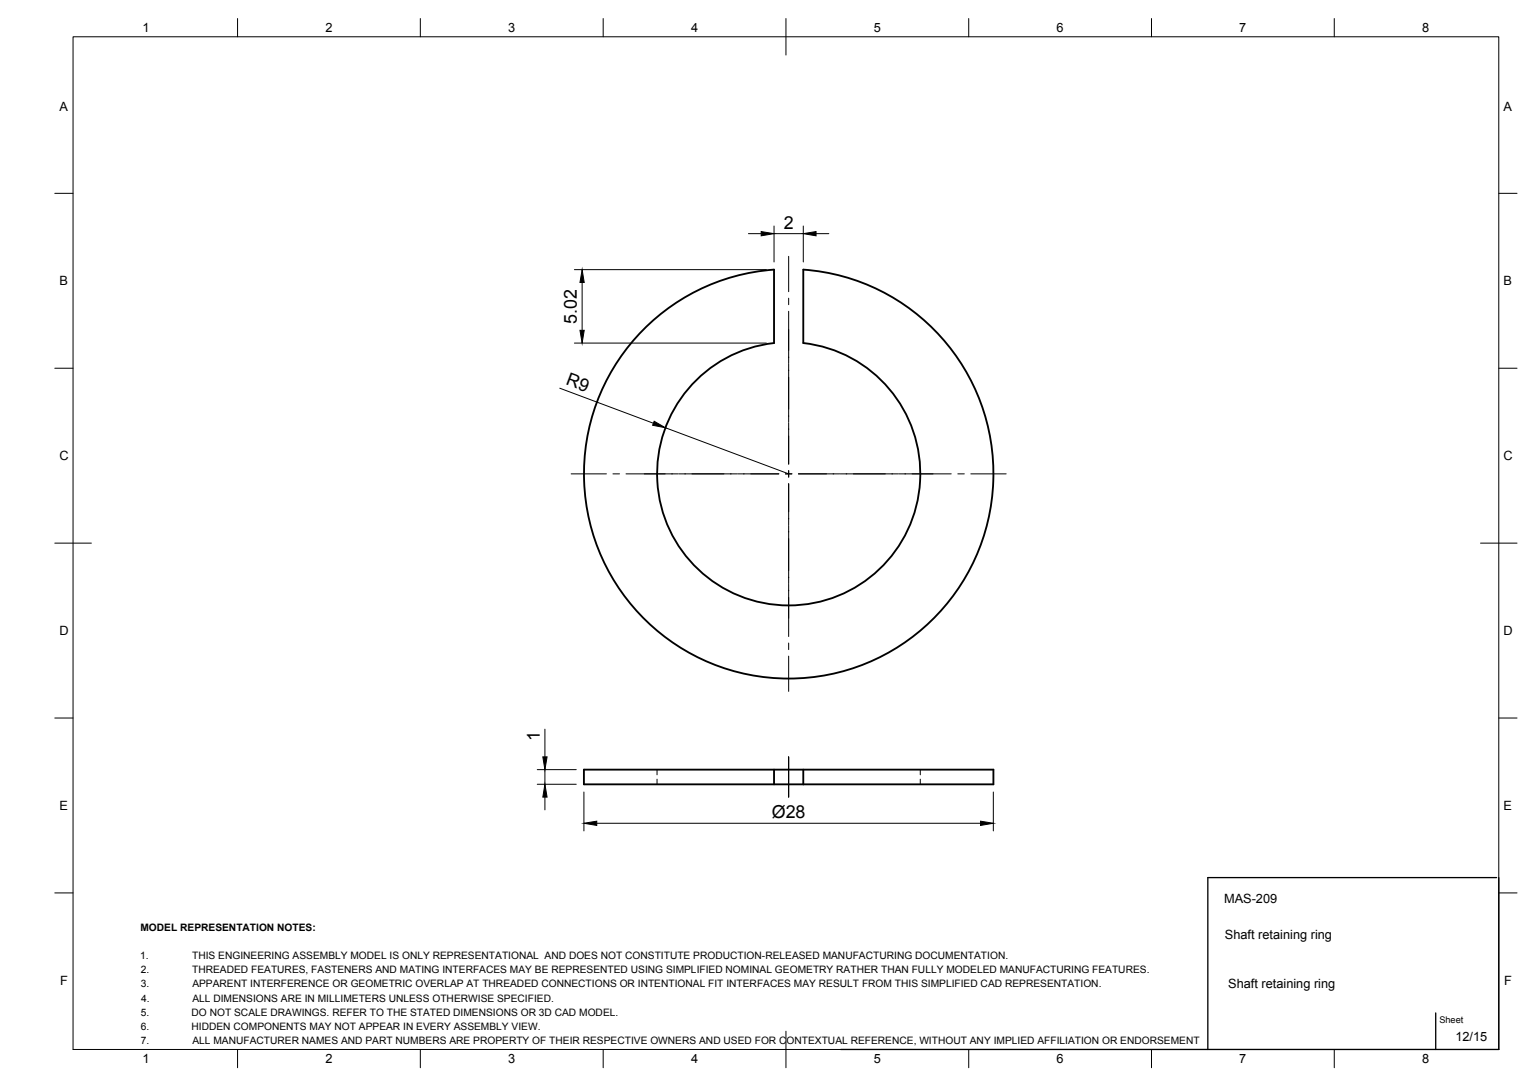
ISO-10303-21;
HEADER;
/* Generated by software containing ST-Developer
 * from STEP Tools, Inc. (www.steptools.com) 
 */

FILE_DESCRIPTION(
/* description */ ('Independent bearing-supported roller-ramp one-way clutch. Six logarit
hmic ramps with plain solid rollers, sprung guided plungers, native Co
il variants, removable shared keepers, rounded parallel key, shaft wit
h complete retaining lips, bronze journal/thrust support and bolted co
vers. Native rotor, roller planar/spin and plunger joints permit manua
l geometric engaged/released inspection. Automatic frictional torque s
witching/contact dynamics are not simulated; no capacity, hardness, fi
t, lubrication, speed, force or life rating. External input driver/cou
pling/anchors outside assembly.'),
/* implementation_level */ '2;1');

FILE_NAME(
/* name */ 'Shaft retaining ring.step',
/* time_stamp */ '2026-11-08T07:04:38-08:00',
/* author */ (''),
/* organization */ (''),
/* preprocessor_version */ 'ST-DEVELOPER v20.2',
/* originating_system */ 'Autodesk Translation Framework v15.17.0.0',
/* authorisation */ '');

FILE_SCHEMA (('AUTOMOTIVE_DESIGN { 1 0 10303 214 3 1 1 }'));
ENDSEC;

DATA;
#10=MECHANICAL_DESIGN_GEOMETRIC_PRESENTATION_REPRESENTATION('',(#311),#99526);
#279=SHAPE_REPRESENTATION_RELATIONSHIP('SRR','None',#99636,#295);
#295=ADVANCED_BREP_SHAPE_REPRESENTATION('',(#327),#99521);
#311=STYLED_ITEM('',(#99722),#327);
#327=MANIFOLD_SOLID_BREP('Body1',#18281);
#585=PLANE('',#19622);
#586=PLANE('',#19623);
#587=PLANE('',#19624);
#588=PLANE('',#19631);
#1578=FACE_OUTER_BOUND('',#2679,.T.);
#1579=FACE_OUTER_BOUND('',#2680,.T.);
#1580=FACE_OUTER_BOUND('',#2681,.T.);
#1581=FACE_OUTER_BOUND('',#2682,.T.);
#1582=FACE_OUTER_BOUND('',#2683,.T.);
#1583=FACE_OUTER_BOUND('',#2684,.T.);
#2679=EDGE_LOOP('',(#16056,#16057,#16058,#16059));
#2680=EDGE_LOOP('',(#16060,#16061,#16062,#16063));
#2681=EDGE_LOOP('',(#16064,#16065,#16066,#16067));
#2682=EDGE_LOOP('',(#16068,#16069,#16070,#16071));
#2683=EDGE_LOOP('',(#16072,#16073,#16074,#16075));
#2684=EDGE_LOOP('',(#16076,#16077,#16078,#16079));
#3088=CIRCLE('',#19625,14.);
#3089=CIRCLE('',#19626,9.);
#3090=CIRCLE('',#19628,9.);
#3091=CIRCLE('',#19630,14.);
#5436=LINE('',#94898,#6340);
#5437=LINE('',#94900,#6341);
#5438=LINE('',#94902,#6342);
#5439=LINE('',#94903,#6343);
#5440=LINE('',#94907,#6344);
#5441=LINE('',#94909,#6345);
#5442=LINE('',#94911,#6346);
#5443=LINE('',#94912,#6347);
#6340=VECTOR('',#22925,10.);
#6341=VECTOR('',#22926,10.);
#6342=VECTOR('',#22927,10.);
#6343=VECTOR('',#22928,10.);
#6344=VECTOR('',#22931,10.);
#6345=VECTOR('',#22932,10.);
#6346=VECTOR('',#22933,10.);
#6347=VECTOR('',#22934,10.);
#8103=VERTEX_POINT('',#94896);
#8104=VERTEX_POINT('',#94897);
#8105=VERTEX_POINT('',#94899);
#8106=VERTEX_POINT('',#94901);
#8107=VERTEX_POINT('',#94905);
#8108=VERTEX_POINT('',#94906);
#8109=VERTEX_POINT('',#94908);
#8110=VERTEX_POINT('',#94910);
#10780=EDGE_CURVE('',#8103,#8104,#5436,.T.);
#10781=EDGE_CURVE('',#8105,#8103,#5437,.T.);
#10782=EDGE_CURVE('',#8106,#8105,#5438,.T.);
#10783=EDGE_CURVE('',#8104,#8106,#5439,.T.);
#10784=EDGE_CURVE('',#8107,#8108,#5440,.T.);
#10785=EDGE_CURVE('',#8109,#8107,#5441,.T.);
#10786=EDGE_CURVE('',#8110,#8109,#5442,.T.);
#10787=EDGE_CURVE('',#8108,#8110,#5443,.T.);
#10788=EDGE_CURVE('',#8105,#8110,#3088,.T.);
#10789=EDGE_CURVE('',#8108,#8103,#3089,.T.);
#10790=EDGE_CURVE('',#8107,#8104,#3090,.T.);
#10791=EDGE_CURVE('',#8106,#8109,#3091,.T.);
#16056=ORIENTED_EDGE('',*,*,#10780,.F.);
#16057=ORIENTED_EDGE('',*,*,#10781,.F.);
#16058=ORIENTED_EDGE('',*,*,#10782,.F.);
#16059=ORIENTED_EDGE('',*,*,#10783,.F.);
#16060=ORIENTED_EDGE('',*,*,#10784,.F.);
#16061=ORIENTED_EDGE('',*,*,#10785,.F.);
#16062=ORIENTED_EDGE('',*,*,#10786,.F.);
#16063=ORIENTED_EDGE('',*,*,#10787,.F.);
#16064=ORIENTED_EDGE('',*,*,#10787,.T.);
#16065=ORIENTED_EDGE('',*,*,#10788,.F.);
#16066=ORIENTED_EDGE('',*,*,#10781,.T.);
#16067=ORIENTED_EDGE('',*,*,#10789,.F.);
#16068=ORIENTED_EDGE('',*,*,#10784,.T.);
#16069=ORIENTED_EDGE('',*,*,#10789,.T.);
#16070=ORIENTED_EDGE('',*,*,#10780,.T.);
#16071=ORIENTED_EDGE('',*,*,#10790,.F.);
#16072=ORIENTED_EDGE('',*,*,#10786,.T.);
#16073=ORIENTED_EDGE('',*,*,#10791,.F.);
#16074=ORIENTED_EDGE('',*,*,#10782,.T.);
#16075=ORIENTED_EDGE('',*,*,#10788,.T.);
#16076=ORIENTED_EDGE('',*,*,#10785,.T.);
#16077=ORIENTED_EDGE('',*,*,#10790,.T.);
#16078=ORIENTED_EDGE('',*,*,#10783,.T.);
#16079=ORIENTED_EDGE('',*,*,#10791,.T.);
#17216=CYLINDRICAL_SURFACE('',#19627,9.);
#17217=CYLINDRICAL_SURFACE('',#19629,14.);
#18176=ADVANCED_FACE('',(#1578),#585,.F.);
#18177=ADVANCED_FACE('',(#1579),#586,.F.);
#18178=ADVANCED_FACE('',(#1580),#587,.F.);
#18179=ADVANCED_FACE('',(#1581),#17216,.F.);
#18180=ADVANCED_FACE('',(#1582),#17217,.T.);
#18181=ADVANCED_FACE('',(#1583),#588,.T.);
#18281=CLOSED_SHELL('',(#18176,#18177,#18178,#18179,#18180,#18181));
#19621=AXIS2_PLACEMENT_3D('',#94894,#22921,#22922);
#19622=AXIS2_PLACEMENT_3D('',#94895,#22923,#22924);
#19623=AXIS2_PLACEMENT_3D('',#94904,#22929,#22930);
#19624=AXIS2_PLACEMENT_3D('',#94913,#22935,#22936);
#19625=AXIS2_PLACEMENT_3D('',#94914,#22937,#22938);
#19626=AXIS2_PLACEMENT_3D('',#94915,#22939,#22940);
#19627=AXIS2_PLACEMENT_3D('',#94916,#22941,#22942);
#19628=AXIS2_PLACEMENT_3D('',#94917,#22943,#22944);
#19629=AXIS2_PLACEMENT_3D('',#94918,#22945,#22946);
#19630=AXIS2_PLACEMENT_3D('',#94919,#22947,#22948);
#19631=AXIS2_PLACEMENT_3D('',#94920,#22949,#22950);
#22921=DIRECTION('axis',(0.,0.,1.));
#22922=DIRECTION('refdir',(1.,0.,0.));
#22923=DIRECTION('center_axis',(-1.,0.,0.));
#22924=DIRECTION('ref_axis',(0.,1.,0.));
#22925=DIRECTION('',(0.,0.,1.));
#22926=DIRECTION('',(0.,-1.,0.));
#22927=DIRECTION('',(0.,0.,-1.));
#22928=DIRECTION('',(0.,1.,0.));
#22929=DIRECTION('center_axis',(1.,0.,0.));
#22930=DIRECTION('ref_axis',(0.,-1.,0.));
#22931=DIRECTION('',(0.,0.,-1.));
#22932=DIRECTION('',(0.,-1.,0.));
#22933=DIRECTION('',(0.,0.,1.));
#22934=DIRECTION('',(0.,1.,0.));
#22935=DIRECTION('center_axis',(0.,0.,1.));
#22936=DIRECTION('ref_axis',(1.,0.,0.));
#22937=DIRECTION('center_axis',(0.,0.,1.));
#22938=DIRECTION('ref_axis',(1.,0.,0.));
#22939=DIRECTION('center_axis',(0.,0.,-1.));
#22940=DIRECTION('ref_axis',(1.,0.,0.));
#22941=DIRECTION('center_axis',(0.,0.,1.));
#22942=DIRECTION('ref_axis',(6.12323399573677E-17,-1.,0.));
#22943=DIRECTION('center_axis',(0.,0.,-1.));
#22944=DIRECTION('ref_axis',(1.,0.,0.));
#22945=DIRECTION('center_axis',(0.,0.,1.));
#22946=DIRECTION('ref_axis',(6.12323399573677E-17,-1.,0.));
#22947=DIRECTION('center_axis',(0.,0.,1.));
#22948=DIRECTION('ref_axis',(1.,0.,0.));
#22949=DIRECTION('center_axis',(0.,0.,1.));
#22950=DIRECTION('ref_axis',(1.,0.,0.));
#94894=CARTESIAN_POINT('',(0.,0.,0.));
#94895=CARTESIAN_POINT('Origin',(-1.,0.,1.));
#94896=CARTESIAN_POINT('',(-1.,8.94427190999916,0.));
#94897=CARTESIAN_POINT('',(-1.,8.94427190999916,1.));
#94898=CARTESIAN_POINT('',(-1.,8.94427190999916,0.));
#94899=CARTESIAN_POINT('',(-1.,13.9642400437689,0.));
#94900=CARTESIAN_POINT('',(-1.,0.,0.));
#94901=CARTESIAN_POINT('',(-1.,13.9642400437689,1.));
#94902=CARTESIAN_POINT('',(-1.,13.9642400437689,0.));
#94903=CARTESIAN_POINT('',(-1.,0.,1.));
#94904=CARTESIAN_POINT('Origin',(1.,28.,1.));
#94905=CARTESIAN_POINT('',(1.,8.94427190999916,1.));
#94906=CARTESIAN_POINT('',(1.,8.94427190999916,0.));
#94907=CARTESIAN_POINT('',(1.,8.94427190999916,0.));
#94908=CARTESIAN_POINT('',(1.,13.9642400437689,1.));
#94909=CARTESIAN_POINT('',(1.,14.,1.));
#94910=CARTESIAN_POINT('',(1.,13.9642400437689,0.));
#94911=CARTESIAN_POINT('',(1.,13.9642400437689,0.));
#94912=CARTESIAN_POINT('',(1.,14.,0.));
#94913=CARTESIAN_POINT('Origin',(0.,0.,0.));
#94914=CARTESIAN_POINT('Origin',(0.,0.,0.));
#94915=CARTESIAN_POINT('Origin',(0.,0.,0.));
#94916=CARTESIAN_POINT('Origin',(0.,0.,0.));
#94917=CARTESIAN_POINT('Origin',(0.,0.,1.));
#94918=CARTESIAN_POINT('Origin',(0.,0.,0.));
#94919=CARTESIAN_POINT('Origin',(0.,0.,1.));
#94920=CARTESIAN_POINT('Origin',(0.,0.,1.));
#99503=UNCERTAINTY_MEASURE_WITH_UNIT(LENGTH_MEASURE(0.01),#99527,
'DISTANCE_ACCURACY_VALUE',
'Maximum model space distance between geometric entities at asserted c
onnectivities');
#99508=UNCERTAINTY_MEASURE_WITH_UNIT(LENGTH_MEASURE(0.01),#99527,
'DISTANCE_ACCURACY_VALUE',
'Maximum model space distance between geometric entities at asserted c
onnectivities');
#99521=(
GEOMETRIC_REPRESENTATION_CONTEXT(3)
GLOBAL_UNCERTAINTY_ASSIGNED_CONTEXT((#99503))
GLOBAL_UNIT_ASSIGNED_CONTEXT((#99527,#99529,#99530))
REPRESENTATION_CONTEXT('','3D')
);
#99526=(
GEOMETRIC_REPRESENTATION_CONTEXT(3)
GLOBAL_UNCERTAINTY_ASSIGNED_CONTEXT((#99508))
GLOBAL_UNIT_ASSIGNED_CONTEXT((#99527,#99529,#99530))
REPRESENTATION_CONTEXT('','3D')
);
#99527=(
LENGTH_UNIT()
NAMED_UNIT(*)
SI_UNIT(.MILLI.,.METRE.)
);
#99529=(
NAMED_UNIT(*)
PLANE_ANGLE_UNIT()
SI_UNIT($,.RADIAN.)
);
#99530=(
NAMED_UNIT(*)
SI_UNIT($,.STERADIAN.)
SOLID_ANGLE_UNIT()
);
#99543=SHAPE_DEFINITION_REPRESENTATION(#99560,#99636);
#99560=PRODUCT_DEFINITION_SHAPE('',$,#99654);
#99636=SHAPE_REPRESENTATION('',(#19621),#99521);
#99641=PRODUCT_DEFINITION_CONTEXT('part definition',#99694,'design');
#99654=PRODUCT_DEFINITION('Shaft retaining ring','Shaft retaining ring',
#99671,#99641);
#99671=PRODUCT_DEFINITION_FORMATION('',$,#99708);
#99694=APPLICATION_CONTEXT(
'Core Data for Automotive Mechanical Design Process');
#99695=PRODUCT_CONTEXT('part definition',#99694,'mechanical');
#99708=PRODUCT('Shaft retaining ring','Shaft retaining ring',$,(#99695));
#99722=PRESENTATION_STYLE_ASSIGNMENT((#99735));
#99735=SURFACE_STYLE_USAGE(.BOTH.,#99748);
#99748=SURFACE_SIDE_STYLE('',(#99761));
#99761=SURFACE_STYLE_FILL_AREA(#99774);
#99774=FILL_AREA_STYLE('Dark gray',(#99787));
#99787=FILL_AREA_STYLE_COLOUR('Dark gray',#99800);
#99800=COLOUR_RGB('Dark gray',0.250980392156863,0.282352941176471,0.32156862745098);
ENDSEC;
END-ISO-10303-21;
